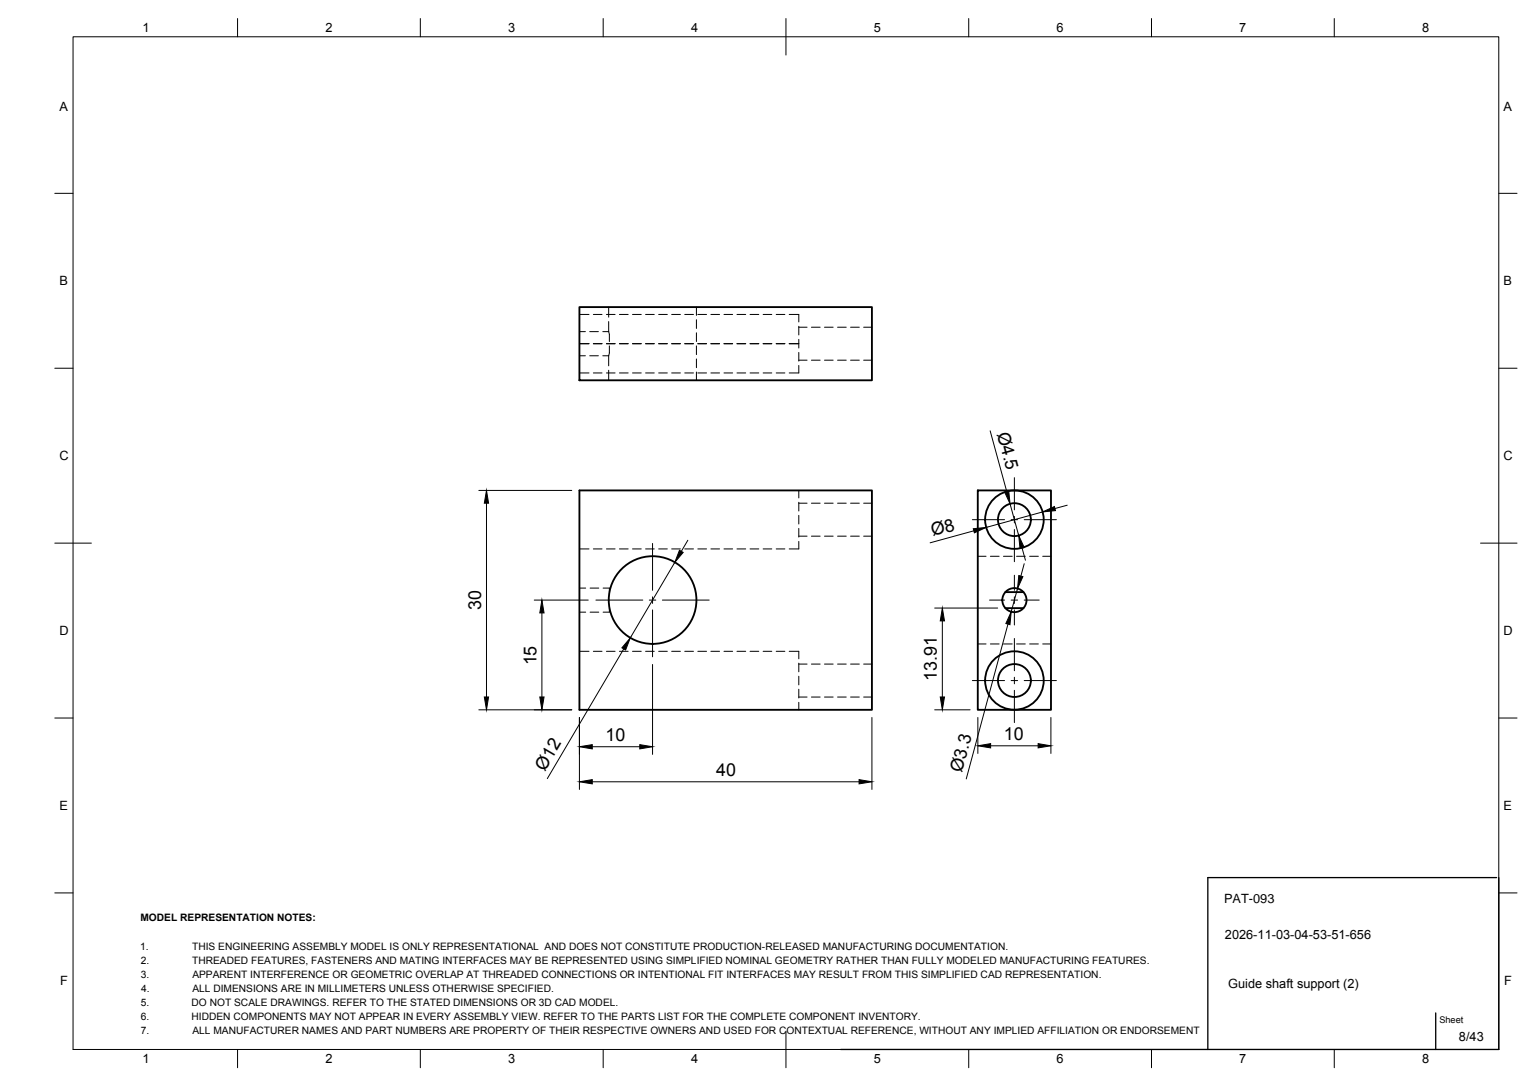
ISO-10303-21;
HEADER;
/* Generated by software containing ST-Developer
 * from STEP Tools, Inc. (www.steptools.com) 
 */

FILE_DESCRIPTION(
/* description */ ('Self-centering screw clamp'),
/* implementation_level */ '2;1');

FILE_NAME(
/* name */ 'Guide shaft support (2).step',
/* time_stamp */ '2026-10-28T03:25:31-07:00',
/* author */ (''),
/* organization */ (''),
/* preprocessor_version */ 'ST-DEVELOPER v20.2',
/* originating_system */ 'Autodesk Translation Framework v15.17.0.0',
/* authorisation */ '');

FILE_SCHEMA (('AUTOMOTIVE_DESIGN { 1 0 10303 214 3 1 1 }'));
ENDSEC;

DATA;
#10=MECHANICAL_DESIGN_GEOMETRIC_PRESENTATION_REPRESENTATION('',(#629),#16799);
#506=B_SPLINE_CURVE_WITH_KNOTS('',3,(#14089,#14090,#14091,#14092,#14093,
#14094),.UNSPECIFIED.,.F.,.F.,(4,2,4),(0.635430324955929,0.687528937234027,
0.750024497760672),.UNSPECIFIED.);
#507=B_SPLINE_CURVE_WITH_KNOTS('',3,(#14098,#14099,#14100,#14101,#14102,
#14103),.UNSPECIFIED.,.F.,.F.,(4,2,4),(0.250008165920224,0.312503726446869,
0.364602338724966),.UNSPECIFIED.);
#508=B_SPLINE_CURVE_WITH_KNOTS('',3,(#14104,#14105,#14106,#14107,#14108,
#14109),.UNSPECIFIED.,.F.,.F.,(4,2,4),(0.135413993115482,0.187512605393579,
0.250008165920224),.UNSPECIFIED.);
#509=B_SPLINE_CURVE_WITH_KNOTS('',3,(#14110,#14111,#14112,#14113,#14114,
#14115),.UNSPECIFIED.,.F.,.F.,(4,2,4),(0.750024497760672,0.812520058287317,
0.864618670565413),.UNSPECIFIED.);
#547=SHAPE_REPRESENTATION_RELATIONSHIP('SRR','None',#17020,#588);
#588=ADVANCED_BREP_SHAPE_REPRESENTATION('',(#677),#16758);
#629=STYLED_ITEM('',(#17326),#677);
#677=MANIFOLD_SOLID_BREP('Body1',#9080);
#756=FACE_BOUND('',#1888,.T.);
#757=FACE_BOUND('',#1891,.T.);
#758=FACE_BOUND('',#1893,.T.);
#759=FACE_BOUND('',#1899,.T.);
#760=FACE_BOUND('',#1902,.T.);
#761=FACE_BOUND('',#1904,.T.);
#762=FACE_BOUND('',#1905,.T.);
#1052=PLANE('',#9715);
#1053=PLANE('',#9720);
#1054=PLANE('',#9724);
#1055=PLANE('',#9729);
#1056=PLANE('',#9731);
#1057=PLANE('',#9739);
#1058=PLANE('',#9740);
#1059=PLANE('',#9741);
#1060=PLANE('',#9742);
#1061=PLANE('',#9743);
#1339=FACE_OUTER_BOUND('',#1881,.T.);
#1340=FACE_OUTER_BOUND('',#1882,.T.);
#1341=FACE_OUTER_BOUND('',#1883,.T.);
#1342=FACE_OUTER_BOUND('',#1884,.T.);
#1343=FACE_OUTER_BOUND('',#1885,.T.);
#1344=FACE_OUTER_BOUND('',#1886,.T.);
#1345=FACE_OUTER_BOUND('',#1887,.T.);
#1346=FACE_OUTER_BOUND('',#1889,.T.);
#1347=FACE_OUTER_BOUND('',#1890,.T.);
#1348=FACE_OUTER_BOUND('',#1892,.T.);
#1349=FACE_OUTER_BOUND('',#1894,.T.);
#1350=FACE_OUTER_BOUND('',#1895,.T.);
#1351=FACE_OUTER_BOUND('',#1896,.T.);
#1352=FACE_OUTER_BOUND('',#1897,.T.);
#1353=FACE_OUTER_BOUND('',#1898,.T.);
#1354=FACE_OUTER_BOUND('',#1900,.T.);
#1355=FACE_OUTER_BOUND('',#1901,.T.);
#1356=FACE_OUTER_BOUND('',#1903,.T.);
#1881=EDGE_LOOP('',(#6439,#6440,#6441,#6442));
#1882=EDGE_LOOP('',(#6443,#6444,#6445,#6446));
#1883=EDGE_LOOP('',(#6447,#6448));
#1884=EDGE_LOOP('',(#6449,#6450,#6451,#6452,#6453,#6454,#6455,#6456,#6457));
#1885=EDGE_LOOP('',(#6458,#6459));
#1886=EDGE_LOOP('',(#6460,#6461,#6462,#6463));
#1887=EDGE_LOOP('',(#6464,#6465));
#1888=EDGE_LOOP('',(#6466));
#1889=EDGE_LOOP('',(#6467,#6468,#6469,#6470));
#1890=EDGE_LOOP('',(#6471,#6472));
#1891=EDGE_LOOP('',(#6473));
#1892=EDGE_LOOP('',(#6474,#6475,#6476,#6477,#6478,#6479,#6480,#6481,#6482,
#6483));
#1893=EDGE_LOOP('',(#6484));
#1894=EDGE_LOOP('',(#6485,#6486,#6487,#6488));
#1895=EDGE_LOOP('',(#6489,#6490,#6491,#6492));
#1896=EDGE_LOOP('',(#6493,#6494,#6495,#6496,#6497,#6498,#6499,#6500,#6501,
#6502,#6503,#6504));
#1897=EDGE_LOOP('',(#6505,#6506,#6507,#6508,#6509,#6510,#6511));
#1898=EDGE_LOOP('',(#6512,#6513,#6514,#6515));
#1899=EDGE_LOOP('',(#6516));
#1900=EDGE_LOOP('',(#6517,#6518,#6519,#6520,#6521,#6522,#6523));
#1901=EDGE_LOOP('',(#6524,#6525,#6526,#6527));
#1902=EDGE_LOOP('',(#6528));
#1903=EDGE_LOOP('',(#6529,#6530,#6531,#6532));
#1904=EDGE_LOOP('',(#6533));
#1905=EDGE_LOOP('',(#6534));
#2679=LINE('',#14066,#3252);
#2680=LINE('',#14070,#3253);
#2681=LINE('',#14075,#3254);
#2682=LINE('',#14079,#3255);
#2683=LINE('',#14084,#3256);
#2684=LINE('',#14117,#3257);
#2685=LINE('',#14120,#3258);
#2686=LINE('',#14123,#3259);
#2687=LINE('',#14130,#3260);
#2688=LINE('',#14138,#3261);
#2689=LINE('',#14139,#3262);
#2690=LINE('',#14141,#3263);
#2691=LINE('',#14143,#3264);
#2692=LINE('',#14144,#3265);
#2693=LINE('',#14145,#3266);
#2694=LINE('',#14149,#3267);
#2695=LINE('',#14153,#3268);
#2696=LINE('',#14157,#3269);
#2697=LINE('',#14159,#3270);
#2698=LINE('',#14164,#3271);
#2699=LINE('',#14165,#3272);
#2700=LINE('',#14166,#3273);
#2701=LINE('',#14169,#3274);
#2702=LINE('',#14170,#3275);
#2703=LINE('',#14173,#3276);
#2704=LINE('',#14174,#3277);
#2705=LINE('',#14176,#3278);
#3252=VECTOR('',#11120,0.4);
#3253=VECTOR('',#11123,1.);
#3254=VECTOR('',#11128,0.4);
#3255=VECTOR('',#11131,1.);
#3256=VECTOR('',#11136,1.);
#3257=VECTOR('',#11143,0.164999999999999);
#3258=VECTOR('',#11148,1.);
#3259=VECTOR('',#11153,1.);
#3260=VECTOR('',#11164,1.);
#3261=VECTOR('',#11173,1.);
#3262=VECTOR('',#11174,1.);
#3263=VECTOR('',#11175,1.);
#3264=VECTOR('',#11176,1.);
#3265=VECTOR('',#11177,1.);
#3266=VECTOR('',#11178,1.);
#3267=VECTOR('',#11183,0.225);
#3268=VECTOR('',#11188,0.225);
#3269=VECTOR('',#11193,0.6);
#3270=VECTOR('',#11194,0.6);
#3271=VECTOR('',#11199,1.);
#3272=VECTOR('',#11200,1.);
#3273=VECTOR('',#11201,1.);
#3274=VECTOR('',#11204,1.);
#3275=VECTOR('',#11205,1.);
#3276=VECTOR('',#11208,1.);
#3277=VECTOR('',#11209,1.);
#3278=VECTOR('',#11212,1.);
#3781=CIRCLE('',#9710,0.4);
#3782=CIRCLE('',#9711,0.4);
#3783=CIRCLE('',#9713,0.4);
#3784=CIRCLE('',#9714,0.4);
#3785=CIRCLE('',#9716,0.164999999999999);
#3786=CIRCLE('',#9718,0.164999999999999);
#3787=CIRCLE('',#9719,0.164999999999999);
#3788=CIRCLE('',#9722,0.4);
#3789=CIRCLE('',#9723,0.4);
#3790=CIRCLE('',#9725,0.225);
#3791=CIRCLE('',#9727,0.4);
#3792=CIRCLE('',#9728,0.4);
#3793=CIRCLE('',#9730,0.225);
#3794=CIRCLE('',#9733,0.225);
#3795=CIRCLE('',#9735,0.225);
#3796=CIRCLE('',#9737,0.6);
#3797=CIRCLE('',#9738,0.6);
#4339=VERTEX_POINT('',#14064);
#4340=VERTEX_POINT('',#14065);
#4341=VERTEX_POINT('',#14067);
#4342=VERTEX_POINT('',#14069);
#4343=VERTEX_POINT('',#14073);
#4344=VERTEX_POINT('',#14074);
#4345=VERTEX_POINT('',#14076);
#4346=VERTEX_POINT('',#14078);
#4347=VERTEX_POINT('',#14082);
#4348=VERTEX_POINT('',#14083);
#4349=VERTEX_POINT('',#14087);
#4350=VERTEX_POINT('',#14088);
#4351=VERTEX_POINT('',#14095);
#4352=VERTEX_POINT('',#14097);
#4353=VERTEX_POINT('',#14116);
#4354=VERTEX_POINT('',#14126);
#4355=VERTEX_POINT('',#14133);
#4356=VERTEX_POINT('',#14136);
#4357=VERTEX_POINT('',#14137);
#4358=VERTEX_POINT('',#14140);
#4359=VERTEX_POINT('',#14142);
#4360=VERTEX_POINT('',#14147);
#4361=VERTEX_POINT('',#14151);
#4362=VERTEX_POINT('',#14155);
#4363=VERTEX_POINT('',#14158);
#4364=VERTEX_POINT('',#14162);
#4365=VERTEX_POINT('',#14163);
#4366=VERTEX_POINT('',#14168);
#4367=VERTEX_POINT('',#14172);
#5144=EDGE_CURVE('',#4339,#4340,#2679,.T.);
#5145=EDGE_CURVE('',#4341,#4339,#3781,.T.);
#5146=EDGE_CURVE('',#4341,#4342,#2680,.T.);
#5147=EDGE_CURVE('',#4340,#4342,#3782,.T.);
#5148=EDGE_CURVE('',#4343,#4344,#2681,.T.);
#5149=EDGE_CURVE('',#4345,#4343,#3783,.T.);
#5150=EDGE_CURVE('',#4345,#4346,#2682,.T.);
#5151=EDGE_CURVE('',#4344,#4346,#3784,.T.);
#5152=EDGE_CURVE('',#4347,#4348,#2683,.T.);
#5153=EDGE_CURVE('',#4347,#4348,#3785,.T.);
#5154=EDGE_CURVE('',#4349,#4350,#506,.T.);
#5155=EDGE_CURVE('',#4351,#4349,#3786,.T.);
#5156=EDGE_CURVE('',#4352,#4351,#507,.T.);
#5157=EDGE_CURVE('',#4348,#4352,#508,.T.);
#5158=EDGE_CURVE('',#4350,#4347,#509,.T.);
#5159=EDGE_CURVE('',#4350,#4353,#2684,.T.);
#5160=EDGE_CURVE('',#4353,#4353,#3787,.T.);
#5161=EDGE_CURVE('',#4351,#4349,#2685,.T.);
#5162=EDGE_CURVE('',#4346,#4344,#3788,.T.);
#5163=EDGE_CURVE('',#4345,#4346,#2686,.T.);
#5164=EDGE_CURVE('',#4343,#4345,#3789,.T.);
#5165=EDGE_CURVE('',#4354,#4354,#3790,.T.);
#5166=EDGE_CURVE('',#4342,#4340,#3791,.T.);
#5167=EDGE_CURVE('',#4341,#4342,#2687,.T.);
#5168=EDGE_CURVE('',#4339,#4341,#3792,.T.);
#5169=EDGE_CURVE('',#4355,#4355,#3793,.T.);
#5170=EDGE_CURVE('',#4356,#4357,#2688,.T.);
#5171=EDGE_CURVE('',#4357,#4346,#2689,.T.);
#5172=EDGE_CURVE('',#4346,#4358,#2690,.T.);
#5173=EDGE_CURVE('',#4358,#4359,#2691,.T.);
#5174=EDGE_CURVE('',#4359,#4342,#2692,.T.);
#5175=EDGE_CURVE('',#4342,#4356,#2693,.T.);
#5176=EDGE_CURVE('',#4360,#4360,#3794,.T.);
#5177=EDGE_CURVE('',#4360,#4354,#2694,.T.);
#5178=EDGE_CURVE('',#4361,#4361,#3795,.T.);
#5179=EDGE_CURVE('',#4361,#4355,#2695,.T.);
#5180=EDGE_CURVE('',#4362,#4362,#3796,.T.);
#5181=EDGE_CURVE('',#4362,#4350,#2696,.T.);
#5182=EDGE_CURVE('',#4352,#4363,#2697,.T.);
#5183=EDGE_CURVE('',#4363,#4363,#3797,.T.);
#5184=EDGE_CURVE('',#4364,#4365,#2698,.T.);
#5185=EDGE_CURVE('',#4365,#4356,#2699,.T.);
#5186=EDGE_CURVE('',#4364,#4359,#2700,.T.);
#5187=EDGE_CURVE('',#4366,#4364,#2701,.T.);
#5188=EDGE_CURVE('',#4366,#4358,#2702,.T.);
#5189=EDGE_CURVE('',#4367,#4366,#2703,.T.);
#5190=EDGE_CURVE('',#4367,#4357,#2704,.T.);
#5191=EDGE_CURVE('',#4365,#4367,#2705,.T.);
#6439=ORIENTED_EDGE('',*,*,#5144,.F.);
#6440=ORIENTED_EDGE('',*,*,#5145,.F.);
#6441=ORIENTED_EDGE('',*,*,#5146,.T.);
#6442=ORIENTED_EDGE('',*,*,#5147,.F.);
#6443=ORIENTED_EDGE('',*,*,#5148,.F.);
#6444=ORIENTED_EDGE('',*,*,#5149,.F.);
#6445=ORIENTED_EDGE('',*,*,#5150,.T.);
#6446=ORIENTED_EDGE('',*,*,#5151,.F.);
#6447=ORIENTED_EDGE('',*,*,#5152,.F.);
#6448=ORIENTED_EDGE('',*,*,#5153,.T.);
#6449=ORIENTED_EDGE('',*,*,#5154,.F.);
#6450=ORIENTED_EDGE('',*,*,#5155,.F.);
#6451=ORIENTED_EDGE('',*,*,#5156,.F.);
#6452=ORIENTED_EDGE('',*,*,#5157,.F.);
#6453=ORIENTED_EDGE('',*,*,#5153,.F.);
#6454=ORIENTED_EDGE('',*,*,#5158,.F.);
#6455=ORIENTED_EDGE('',*,*,#5159,.T.);
#6456=ORIENTED_EDGE('',*,*,#5160,.F.);
#6457=ORIENTED_EDGE('',*,*,#5159,.F.);
#6458=ORIENTED_EDGE('',*,*,#5161,.F.);
#6459=ORIENTED_EDGE('',*,*,#5155,.T.);
#6460=ORIENTED_EDGE('',*,*,#5148,.T.);
#6461=ORIENTED_EDGE('',*,*,#5162,.F.);
#6462=ORIENTED_EDGE('',*,*,#5163,.F.);
#6463=ORIENTED_EDGE('',*,*,#5164,.F.);
#6464=ORIENTED_EDGE('',*,*,#5149,.T.);
#6465=ORIENTED_EDGE('',*,*,#5164,.T.);
#6466=ORIENTED_EDGE('',*,*,#5165,.F.);
#6467=ORIENTED_EDGE('',*,*,#5144,.T.);
#6468=ORIENTED_EDGE('',*,*,#5166,.F.);
#6469=ORIENTED_EDGE('',*,*,#5167,.F.);
#6470=ORIENTED_EDGE('',*,*,#5168,.F.);
#6471=ORIENTED_EDGE('',*,*,#5145,.T.);
#6472=ORIENTED_EDGE('',*,*,#5168,.T.);
#6473=ORIENTED_EDGE('',*,*,#5169,.F.);
#6474=ORIENTED_EDGE('',*,*,#5170,.T.);
#6475=ORIENTED_EDGE('',*,*,#5171,.T.);
#6476=ORIENTED_EDGE('',*,*,#5162,.T.);
#6477=ORIENTED_EDGE('',*,*,#5151,.T.);
#6478=ORIENTED_EDGE('',*,*,#5172,.T.);
#6479=ORIENTED_EDGE('',*,*,#5173,.T.);
#6480=ORIENTED_EDGE('',*,*,#5174,.T.);
#6481=ORIENTED_EDGE('',*,*,#5166,.T.);
#6482=ORIENTED_EDGE('',*,*,#5147,.T.);
#6483=ORIENTED_EDGE('',*,*,#5175,.T.);
#6484=ORIENTED_EDGE('',*,*,#5160,.T.);
#6485=ORIENTED_EDGE('',*,*,#5176,.F.);
#6486=ORIENTED_EDGE('',*,*,#5177,.T.);
#6487=ORIENTED_EDGE('',*,*,#5165,.T.);
#6488=ORIENTED_EDGE('',*,*,#5177,.F.);
#6489=ORIENTED_EDGE('',*,*,#5178,.F.);
#6490=ORIENTED_EDGE('',*,*,#5179,.T.);
#6491=ORIENTED_EDGE('',*,*,#5169,.T.);
#6492=ORIENTED_EDGE('',*,*,#5179,.F.);
#6493=ORIENTED_EDGE('',*,*,#5180,.F.);
#6494=ORIENTED_EDGE('',*,*,#5181,.T.);
#6495=ORIENTED_EDGE('',*,*,#5158,.T.);
#6496=ORIENTED_EDGE('',*,*,#5152,.T.);
#6497=ORIENTED_EDGE('',*,*,#5157,.T.);
#6498=ORIENTED_EDGE('',*,*,#5182,.T.);
#6499=ORIENTED_EDGE('',*,*,#5183,.F.);
#6500=ORIENTED_EDGE('',*,*,#5182,.F.);
#6501=ORIENTED_EDGE('',*,*,#5156,.T.);
#6502=ORIENTED_EDGE('',*,*,#5161,.T.);
#6503=ORIENTED_EDGE('',*,*,#5154,.T.);
#6504=ORIENTED_EDGE('',*,*,#5181,.F.);
#6505=ORIENTED_EDGE('',*,*,#5184,.T.);
#6506=ORIENTED_EDGE('',*,*,#5185,.T.);
#6507=ORIENTED_EDGE('',*,*,#5175,.F.);
#6508=ORIENTED_EDGE('',*,*,#5146,.F.);
#6509=ORIENTED_EDGE('',*,*,#5167,.T.);
#6510=ORIENTED_EDGE('',*,*,#5174,.F.);
#6511=ORIENTED_EDGE('',*,*,#5186,.F.);
#6512=ORIENTED_EDGE('',*,*,#5187,.T.);
#6513=ORIENTED_EDGE('',*,*,#5186,.T.);
#6514=ORIENTED_EDGE('',*,*,#5173,.F.);
#6515=ORIENTED_EDGE('',*,*,#5188,.F.);
#6516=ORIENTED_EDGE('',*,*,#5183,.T.);
#6517=ORIENTED_EDGE('',*,*,#5189,.T.);
#6518=ORIENTED_EDGE('',*,*,#5188,.T.);
#6519=ORIENTED_EDGE('',*,*,#5172,.F.);
#6520=ORIENTED_EDGE('',*,*,#5150,.F.);
#6521=ORIENTED_EDGE('',*,*,#5163,.T.);
#6522=ORIENTED_EDGE('',*,*,#5171,.F.);
#6523=ORIENTED_EDGE('',*,*,#5190,.F.);
#6524=ORIENTED_EDGE('',*,*,#5191,.T.);
#6525=ORIENTED_EDGE('',*,*,#5190,.T.);
#6526=ORIENTED_EDGE('',*,*,#5170,.F.);
#6527=ORIENTED_EDGE('',*,*,#5185,.F.);
#6528=ORIENTED_EDGE('',*,*,#5180,.T.);
#6529=ORIENTED_EDGE('',*,*,#5191,.F.);
#6530=ORIENTED_EDGE('',*,*,#5184,.F.);
#6531=ORIENTED_EDGE('',*,*,#5187,.F.);
#6532=ORIENTED_EDGE('',*,*,#5189,.F.);
#6533=ORIENTED_EDGE('',*,*,#5176,.T.);
#6534=ORIENTED_EDGE('',*,*,#5178,.T.);
#8385=CYLINDRICAL_SURFACE('',#9709,0.4);
#8386=CYLINDRICAL_SURFACE('',#9712,0.4);
#8387=CYLINDRICAL_SURFACE('',#9717,0.164999999999999);
#8388=CYLINDRICAL_SURFACE('',#9721,0.4);
#8389=CYLINDRICAL_SURFACE('',#9726,0.4);
#8390=CYLINDRICAL_SURFACE('',#9732,0.225);
#8391=CYLINDRICAL_SURFACE('',#9734,0.225);
#8392=CYLINDRICAL_SURFACE('',#9736,0.6);
#8637=ADVANCED_FACE('',(#1339),#8385,.F.);
#8638=ADVANCED_FACE('',(#1340),#8386,.F.);
#8639=ADVANCED_FACE('',(#1341),#1052,.T.);
#8640=ADVANCED_FACE('',(#1342),#8387,.F.);
#8641=ADVANCED_FACE('',(#1343),#1053,.T.);
#8642=ADVANCED_FACE('',(#1344),#8388,.F.);
#8643=ADVANCED_FACE('',(#1345,#756),#1054,.T.);
#8644=ADVANCED_FACE('',(#1346),#8389,.F.);
#8645=ADVANCED_FACE('',(#1347,#757),#1055,.T.);
#8646=ADVANCED_FACE('',(#1348,#758),#1056,.T.);
#8647=ADVANCED_FACE('',(#1349),#8390,.F.);
#8648=ADVANCED_FACE('',(#1350),#8391,.F.);
#8649=ADVANCED_FACE('',(#1351),#8392,.F.);
#8650=ADVANCED_FACE('',(#1352),#1057,.T.);
#8651=ADVANCED_FACE('',(#1353,#759),#1058,.T.);
#8652=ADVANCED_FACE('',(#1354),#1059,.T.);
#8653=ADVANCED_FACE('',(#1355,#760),#1060,.T.);
#8654=ADVANCED_FACE('',(#1356,#761,#762),#1061,.F.);
#9080=CLOSED_SHELL('',(#8637,#8638,#8639,#8640,#8641,#8642,#8643,#8644,
#8645,#8646,#8647,#8648,#8649,#8650,#8651,#8652,#8653,#8654));
#9708=AXIS2_PLACEMENT_3D('',#14062,#11116,#11117);
#9709=AXIS2_PLACEMENT_3D('',#14063,#11118,#11119);
#9710=AXIS2_PLACEMENT_3D('',#14068,#11121,#11122);
#9711=AXIS2_PLACEMENT_3D('',#14071,#11124,#11125);
#9712=AXIS2_PLACEMENT_3D('',#14072,#11126,#11127);
#9713=AXIS2_PLACEMENT_3D('',#14077,#11129,#11130);
#9714=AXIS2_PLACEMENT_3D('',#14080,#11132,#11133);
#9715=AXIS2_PLACEMENT_3D('',#14081,#11134,#11135);
#9716=AXIS2_PLACEMENT_3D('',#14085,#11137,#11138);
#9717=AXIS2_PLACEMENT_3D('',#14086,#11139,#11140);
#9718=AXIS2_PLACEMENT_3D('',#14096,#11141,#11142);
#9719=AXIS2_PLACEMENT_3D('',#14118,#11144,#11145);
#9720=AXIS2_PLACEMENT_3D('',#14119,#11146,#11147);
#9721=AXIS2_PLACEMENT_3D('',#14121,#11149,#11150);
#9722=AXIS2_PLACEMENT_3D('',#14122,#11151,#11152);
#9723=AXIS2_PLACEMENT_3D('',#14124,#11154,#11155);
#9724=AXIS2_PLACEMENT_3D('',#14125,#11156,#11157);
#9725=AXIS2_PLACEMENT_3D('',#14127,#11158,#11159);
#9726=AXIS2_PLACEMENT_3D('',#14128,#11160,#11161);
#9727=AXIS2_PLACEMENT_3D('',#14129,#11162,#11163);
#9728=AXIS2_PLACEMENT_3D('',#14131,#11165,#11166);
#9729=AXIS2_PLACEMENT_3D('',#14132,#11167,#11168);
#9730=AXIS2_PLACEMENT_3D('',#14134,#11169,#11170);
#9731=AXIS2_PLACEMENT_3D('',#14135,#11171,#11172);
#9732=AXIS2_PLACEMENT_3D('',#14146,#11179,#11180);
#9733=AXIS2_PLACEMENT_3D('',#14148,#11181,#11182);
#9734=AXIS2_PLACEMENT_3D('',#14150,#11184,#11185);
#9735=AXIS2_PLACEMENT_3D('',#14152,#11186,#11187);
#9736=AXIS2_PLACEMENT_3D('',#14154,#11189,#11190);
#9737=AXIS2_PLACEMENT_3D('',#14156,#11191,#11192);
#9738=AXIS2_PLACEMENT_3D('',#14160,#11195,#11196);
#9739=AXIS2_PLACEMENT_3D('',#14161,#11197,#11198);
#9740=AXIS2_PLACEMENT_3D('',#14167,#11202,#11203);
#9741=AXIS2_PLACEMENT_3D('',#14171,#11206,#11207);
#9742=AXIS2_PLACEMENT_3D('',#14175,#11210,#11211);
#9743=AXIS2_PLACEMENT_3D('',#14177,#11213,#11214);
#11116=DIRECTION('axis',(0.,0.,1.));
#11117=DIRECTION('refdir',(1.,0.,0.));
#11118=DIRECTION('center_axis',(0.,0.,1.));
#11119=DIRECTION('ref_axis',(1.,0.,0.));
#11120=DIRECTION('',(0.,0.,1.));
#11121=DIRECTION('center_axis',(0.,0.,1.));
#11122=DIRECTION('ref_axis',(1.,0.,0.));
#11123=DIRECTION('',(0.,0.,1.));
#11124=DIRECTION('center_axis',(0.,0.,-1.));
#11125=DIRECTION('ref_axis',(1.,0.,0.));
#11126=DIRECTION('center_axis',(0.,0.,1.));
#11127=DIRECTION('ref_axis',(1.,0.,0.));
#11128=DIRECTION('',(0.,0.,1.));
#11129=DIRECTION('center_axis',(0.,0.,1.));
#11130=DIRECTION('ref_axis',(1.,0.,0.));
#11131=DIRECTION('',(0.,0.,1.));
#11132=DIRECTION('center_axis',(0.,0.,-1.));
#11133=DIRECTION('ref_axis',(1.,0.,0.));
#11134=DIRECTION('center_axis',(0.,0.,1.));
#11135=DIRECTION('ref_axis',(1.,0.,0.));
#11136=DIRECTION('',(1.,0.,0.));
#11137=DIRECTION('center_axis',(0.,0.,1.));
#11138=DIRECTION('ref_axis',(1.,0.,0.));
#11139=DIRECTION('center_axis',(0.,0.,1.));
#11140=DIRECTION('ref_axis',(1.,0.,0.));
#11141=DIRECTION('center_axis',(0.,0.,1.));
#11142=DIRECTION('ref_axis',(1.,0.,0.));
#11143=DIRECTION('',(0.,0.,1.));
#11144=DIRECTION('center_axis',(0.,0.,-1.));
#11145=DIRECTION('ref_axis',(1.,0.,0.));
#11146=DIRECTION('center_axis',(0.,0.,1.));
#11147=DIRECTION('ref_axis',(1.,0.,0.));
#11148=DIRECTION('',(-1.,0.,0.));
#11149=DIRECTION('center_axis',(0.,0.,1.));
#11150=DIRECTION('ref_axis',(1.,0.,0.));
#11151=DIRECTION('center_axis',(0.,0.,-1.));
#11152=DIRECTION('ref_axis',(1.,0.,0.));
#11153=DIRECTION('',(0.,0.,1.));
#11154=DIRECTION('center_axis',(0.,0.,1.));
#11155=DIRECTION('ref_axis',(1.,0.,0.));
#11156=DIRECTION('center_axis',(0.,0.,1.));
#11157=DIRECTION('ref_axis',(1.,0.,0.));
#11158=DIRECTION('center_axis',(0.,0.,1.));
#11159=DIRECTION('ref_axis',(1.,0.,0.));
#11160=DIRECTION('center_axis',(0.,0.,1.));
#11161=DIRECTION('ref_axis',(1.,0.,0.));
#11162=DIRECTION('center_axis',(0.,0.,-1.));
#11163=DIRECTION('ref_axis',(1.,0.,0.));
#11164=DIRECTION('',(0.,0.,1.));
#11165=DIRECTION('center_axis',(0.,0.,1.));
#11166=DIRECTION('ref_axis',(1.,0.,0.));
#11167=DIRECTION('center_axis',(0.,0.,1.));
#11168=DIRECTION('ref_axis',(1.,0.,0.));
#11169=DIRECTION('center_axis',(0.,0.,1.));
#11170=DIRECTION('ref_axis',(1.,0.,0.));
#11171=DIRECTION('center_axis',(0.,0.,1.));
#11172=DIRECTION('ref_axis',(1.,0.,0.));
#11173=DIRECTION('',(0.,-1.,0.));
#11174=DIRECTION('',(1.,0.,0.));
#11175=DIRECTION('',(1.,0.,0.));
#11176=DIRECTION('',(0.,1.,0.));
#11177=DIRECTION('',(-1.,0.,0.));
#11178=DIRECTION('',(-1.,0.,0.));
#11179=DIRECTION('center_axis',(0.,0.,1.));
#11180=DIRECTION('ref_axis',(1.,0.,0.));
#11181=DIRECTION('center_axis',(0.,0.,1.));
#11182=DIRECTION('ref_axis',(1.,0.,0.));
#11183=DIRECTION('',(0.,0.,1.));
#11184=DIRECTION('center_axis',(0.,0.,1.));
#11185=DIRECTION('ref_axis',(1.,0.,0.));
#11186=DIRECTION('center_axis',(0.,0.,1.));
#11187=DIRECTION('ref_axis',(1.,0.,0.));
#11188=DIRECTION('',(0.,0.,1.));
#11189=DIRECTION('center_axis',(1.,0.,0.));
#11190=DIRECTION('ref_axis',(0.,0.,-1.));
#11191=DIRECTION('center_axis',(1.,0.,0.));
#11192=DIRECTION('ref_axis',(0.,0.,-1.));
#11193=DIRECTION('',(1.,0.,0.));
#11194=DIRECTION('',(1.,0.,0.));
#11195=DIRECTION('center_axis',(-1.,0.,0.));
#11196=DIRECTION('ref_axis',(0.,0.,-1.));
#11197=DIRECTION('center_axis',(0.,1.,0.));
#11198=DIRECTION('ref_axis',(-1.,0.,0.));
#11199=DIRECTION('',(-1.,0.,0.));
#11200=DIRECTION('',(0.,0.,1.));
#11201=DIRECTION('',(0.,0.,1.));
#11202=DIRECTION('center_axis',(1.,0.,0.));
#11203=DIRECTION('ref_axis',(0.,1.,0.));
#11204=DIRECTION('',(0.,1.,0.));
#11205=DIRECTION('',(0.,0.,1.));
#11206=DIRECTION('center_axis',(0.,-1.,0.));
#11207=DIRECTION('ref_axis',(1.,0.,0.));
#11208=DIRECTION('',(1.,0.,0.));
#11209=DIRECTION('',(0.,0.,1.));
#11210=DIRECTION('center_axis',(-1.,0.,0.));
#11211=DIRECTION('ref_axis',(0.,-1.,0.));
#11212=DIRECTION('',(0.,-1.,0.));
#11213=DIRECTION('center_axis',(0.,0.,1.));
#11214=DIRECTION('ref_axis',(1.,0.,0.));
#14062=CARTESIAN_POINT('',(0.,0.,0.));
#14063=CARTESIAN_POINT('Origin',(-13.5,4.1,2.));
#14064=CARTESIAN_POINT('',(-13.9,4.1,2.));
#14065=CARTESIAN_POINT('',(-13.9,4.1,5.));
#14066=CARTESIAN_POINT('',(-13.9,4.1,2.));
#14067=CARTESIAN_POINT('',(-13.5,4.5,2.));
#14068=CARTESIAN_POINT('Origin',(-13.5,4.1,2.));
#14069=CARTESIAN_POINT('',(-13.5,4.5,5.));
#14070=CARTESIAN_POINT('',(-13.5,4.5,2.));
#14071=CARTESIAN_POINT('Origin',(-13.5,4.1,5.));
#14072=CARTESIAN_POINT('Origin',(-13.5,1.9,2.));
#14073=CARTESIAN_POINT('',(-13.9,1.9,2.));
#14074=CARTESIAN_POINT('',(-13.9,1.9,5.));
#14075=CARTESIAN_POINT('',(-13.9,1.9,2.));
#14076=CARTESIAN_POINT('',(-13.5,1.5,2.));
#14077=CARTESIAN_POINT('Origin',(-13.5,1.9,2.));
#14078=CARTESIAN_POINT('',(-13.5,1.5,5.));
#14079=CARTESIAN_POINT('',(-13.5,1.5,2.));
#14080=CARTESIAN_POINT('Origin',(-13.5,1.9,5.));
#14081=CARTESIAN_POINT('Origin',(-13.5,3.,4.59));
#14082=CARTESIAN_POINT('',(-13.6237941840314,2.89091287885364,4.59));
#14083=CARTESIAN_POINT('',(-13.3762058159686,2.89091287885364,4.59));
#14084=CARTESIAN_POINT('',(-14.1,2.89091287885364,4.59));
#14085=CARTESIAN_POINT('Origin',(-13.5,3.,4.59));
#14086=CARTESIAN_POINT('Origin',(-13.5,3.,4.59));
#14087=CARTESIAN_POINT('',(-13.6237941840314,3.10908712114636,4.59));
#14088=CARTESIAN_POINT('',(-13.665,3.,4.6));
#14089=CARTESIAN_POINT('Ctrl Pts',(-13.6237941840314,3.10908712114636,4.59));
#14090=CARTESIAN_POINT('Ctrl Pts',(-13.6353991351895,3.09591759715261,4.59243495840567));
#14091=CARTESIAN_POINT('Ctrl Pts',(-13.6453456436582,3.08022344943772,4.59485638705045));
#14092=CARTESIAN_POINT('Ctrl Pts',(-13.660814864634,3.04298016596019,4.59880705606552));
#14093=CARTESIAN_POINT('Ctrl Pts',(-13.665,3.02083185350888,4.6));
#14094=CARTESIAN_POINT('Ctrl Pts',(-13.665,3.,4.6));
#14095=CARTESIAN_POINT('',(-13.3762058159686,3.10908712114636,4.59));
#14096=CARTESIAN_POINT('Origin',(-13.5,3.,4.59));
#14097=CARTESIAN_POINT('',(-13.335,3.,4.6));
#14098=CARTESIAN_POINT('Ctrl Pts',(-13.335,3.,4.6));
#14099=CARTESIAN_POINT('Ctrl Pts',(-13.335,3.02083185350888,4.6));
#14100=CARTESIAN_POINT('Ctrl Pts',(-13.339185135366,3.04298016596019,4.59880705606552));
#14101=CARTESIAN_POINT('Ctrl Pts',(-13.3546543563418,3.08022344943772,4.59485638705045));
#14102=CARTESIAN_POINT('Ctrl Pts',(-13.3646008648105,3.09591759715261,4.59243495840567));
#14103=CARTESIAN_POINT('Ctrl Pts',(-13.3762058159686,3.10908712114636,4.59));
#14104=CARTESIAN_POINT('Ctrl Pts',(-13.3762058159686,2.89091287885364,4.59));
#14105=CARTESIAN_POINT('Ctrl Pts',(-13.3646008648105,2.90408240284739,4.59243495840567));
#14106=CARTESIAN_POINT('Ctrl Pts',(-13.3546543563418,2.91977655056228,4.59485638705045));
#14107=CARTESIAN_POINT('Ctrl Pts',(-13.339185135366,2.95701983403981,4.59880705606552));
#14108=CARTESIAN_POINT('Ctrl Pts',(-13.335,2.97916814649112,4.6));
#14109=CARTESIAN_POINT('Ctrl Pts',(-13.335,3.,4.6));
#14110=CARTESIAN_POINT('Ctrl Pts',(-13.665,3.,4.6));
#14111=CARTESIAN_POINT('Ctrl Pts',(-13.665,2.97916814649112,4.6));
#14112=CARTESIAN_POINT('Ctrl Pts',(-13.660814864634,2.95701983403981,4.59880705606552));
#14113=CARTESIAN_POINT('Ctrl Pts',(-13.6453456436582,2.91977655056228,4.59485638705045));
#14114=CARTESIAN_POINT('Ctrl Pts',(-13.6353991351895,2.90408240284739,4.59243495840567));
#14115=CARTESIAN_POINT('Ctrl Pts',(-13.6237941840314,2.89091287885364,4.59));
#14116=CARTESIAN_POINT('',(-13.665,3.,5.));
#14117=CARTESIAN_POINT('',(-13.665,3.,4.59));
#14118=CARTESIAN_POINT('Origin',(-13.5,3.,5.));
#14119=CARTESIAN_POINT('Origin',(-13.5,3.,4.59));
#14120=CARTESIAN_POINT('',(-14.1,3.10908712114636,4.59));
#14121=CARTESIAN_POINT('Origin',(-13.5,1.9,2.));
#14122=CARTESIAN_POINT('Origin',(-13.5,1.9,5.));
#14123=CARTESIAN_POINT('',(-13.5,1.5,2.));
#14124=CARTESIAN_POINT('Origin',(-13.5,1.9,2.));
#14125=CARTESIAN_POINT('Origin',(-13.5,1.9,2.));
#14126=CARTESIAN_POINT('',(-13.725,1.9,2.));
#14127=CARTESIAN_POINT('Origin',(-13.5,1.9,2.));
#14128=CARTESIAN_POINT('Origin',(-13.5,4.1,2.));
#14129=CARTESIAN_POINT('Origin',(-13.5,4.1,5.));
#14130=CARTESIAN_POINT('',(-13.5,4.5,2.));
#14131=CARTESIAN_POINT('Origin',(-13.5,4.1,2.));
#14132=CARTESIAN_POINT('Origin',(-13.5,4.1,2.));
#14133=CARTESIAN_POINT('',(-13.725,4.1,2.));
#14134=CARTESIAN_POINT('Origin',(-13.5,4.1,2.));
#14135=CARTESIAN_POINT('Origin',(-13.5,3.,5.));
#14136=CARTESIAN_POINT('',(-14.,4.5,5.));
#14137=CARTESIAN_POINT('',(-14.,1.5,5.));
#14138=CARTESIAN_POINT('',(-14.,4.5,5.));
#14139=CARTESIAN_POINT('',(-14.,1.5,5.));
#14140=CARTESIAN_POINT('',(-13.,1.5,5.));
#14141=CARTESIAN_POINT('',(-14.,1.5,5.));
#14142=CARTESIAN_POINT('',(-13.,4.5,5.));
#14143=CARTESIAN_POINT('',(-13.,1.5,5.));
#14144=CARTESIAN_POINT('',(-13.,4.5,5.));
#14145=CARTESIAN_POINT('',(-13.,4.5,5.));
#14146=CARTESIAN_POINT('Origin',(-13.5,1.9,0.9));
#14147=CARTESIAN_POINT('',(-13.725,1.9,1.));
#14148=CARTESIAN_POINT('Origin',(-13.5,1.9,1.));
#14149=CARTESIAN_POINT('',(-13.725,1.9,0.9));
#14150=CARTESIAN_POINT('Origin',(-13.5,4.1,0.9));
#14151=CARTESIAN_POINT('',(-13.725,4.1,1.));
#14152=CARTESIAN_POINT('Origin',(-13.5,4.1,1.));
#14153=CARTESIAN_POINT('',(-13.725,4.1,0.9));
#14154=CARTESIAN_POINT('Origin',(-14.1,3.,4.));
#14155=CARTESIAN_POINT('',(-14.,3.,4.6));
#14156=CARTESIAN_POINT('Origin',(-14.,3.,4.));
#14157=CARTESIAN_POINT('',(-14.1,3.,4.6));
#14158=CARTESIAN_POINT('',(-13.,3.,4.6));
#14159=CARTESIAN_POINT('',(-14.1,3.,4.6));
#14160=CARTESIAN_POINT('Origin',(-13.,3.,4.));
#14161=CARTESIAN_POINT('Origin',(-13.,4.5,1.));
#14162=CARTESIAN_POINT('',(-13.,4.5,1.));
#14163=CARTESIAN_POINT('',(-14.,4.5,1.));
#14164=CARTESIAN_POINT('',(-13.,4.5,1.));
#14165=CARTESIAN_POINT('',(-14.,4.5,1.));
#14166=CARTESIAN_POINT('',(-13.,4.5,1.));
#14167=CARTESIAN_POINT('Origin',(-13.,1.5,1.));
#14168=CARTESIAN_POINT('',(-13.,1.5,1.));
#14169=CARTESIAN_POINT('',(-13.,1.5,1.));
#14170=CARTESIAN_POINT('',(-13.,1.5,1.));
#14171=CARTESIAN_POINT('Origin',(-14.,1.5,1.));
#14172=CARTESIAN_POINT('',(-14.,1.5,1.));
#14173=CARTESIAN_POINT('',(-14.,1.5,1.));
#14174=CARTESIAN_POINT('',(-14.,1.5,1.));
#14175=CARTESIAN_POINT('Origin',(-14.,4.5,1.));
#14176=CARTESIAN_POINT('',(-14.,4.5,1.));
#14177=CARTESIAN_POINT('Origin',(-13.5,3.,1.));
#16709=UNCERTAINTY_MEASURE_WITH_UNIT(LENGTH_MEASURE(0.001),#16800,
'DISTANCE_ACCURACY_VALUE',
'Maximum model space distance between geometric entities at asserted c
onnectivities');
#16750=UNCERTAINTY_MEASURE_WITH_UNIT(LENGTH_MEASURE(0.001),#16800,
'DISTANCE_ACCURACY_VALUE',
'Maximum model space distance between geometric entities at asserted c
onnectivities');
#16758=(
GEOMETRIC_REPRESENTATION_CONTEXT(3)
GLOBAL_UNCERTAINTY_ASSIGNED_CONTEXT((#16709))
GLOBAL_UNIT_ASSIGNED_CONTEXT((#16800,#16802,#16803))
REPRESENTATION_CONTEXT('','3D')
);
#16799=(
GEOMETRIC_REPRESENTATION_CONTEXT(3)
GLOBAL_UNCERTAINTY_ASSIGNED_CONTEXT((#16750))
GLOBAL_UNIT_ASSIGNED_CONTEXT((#16800,#16802,#16803))
REPRESENTATION_CONTEXT('','3D')
);
#16800=(
LENGTH_UNIT()
NAMED_UNIT(*)
SI_UNIT(.CENTI.,.METRE.)
);
#16802=(
NAMED_UNIT(*)
PLANE_ANGLE_UNIT()
SI_UNIT($,.RADIAN.)
);
#16803=(
NAMED_UNIT(*)
SI_UNIT($,.STERADIAN.)
SOLID_ANGLE_UNIT()
);
#16811=SHAPE_DEFINITION_REPRESENTATION(#16859,#17020);
#16859=PRODUCT_DEFINITION_SHAPE('',$,#17069);
#17020=SHAPE_REPRESENTATION('',(#9708),#16758);
#17061=PRODUCT_DEFINITION_CONTEXT('part definition',#17207,'design');
#17069=PRODUCT_DEFINITION('Guide shaft support (2)',
'Guide shaft support (2)',#17117,#17061);
#17117=PRODUCT_DEFINITION_FORMATION('',$,#17216);
#17207=APPLICATION_CONTEXT(
'Core Data for Automotive Mechanical Design Process');
#17208=PRODUCT_CONTEXT('part definition',#17207,'mechanical');
#17216=PRODUCT('Guide shaft support (2)','Guide shaft support (2)',
'Guide shaft support (2)',(#17208));
#17320=COLOUR_RGB('Grey',0.48,0.52,0.57);
#17321=FILL_AREA_STYLE_COLOUR('',#17320);
#17322=FILL_AREA_STYLE('',(#17321));
#17323=SURFACE_STYLE_FILL_AREA(#17322);
#17324=SURFACE_SIDE_STYLE('',(#17323));
#17325=SURFACE_STYLE_USAGE(.BOTH.,#17324);
#17326=PRESENTATION_STYLE_ASSIGNMENT((#17325));
ENDSEC;
END-ISO-10303-21;
